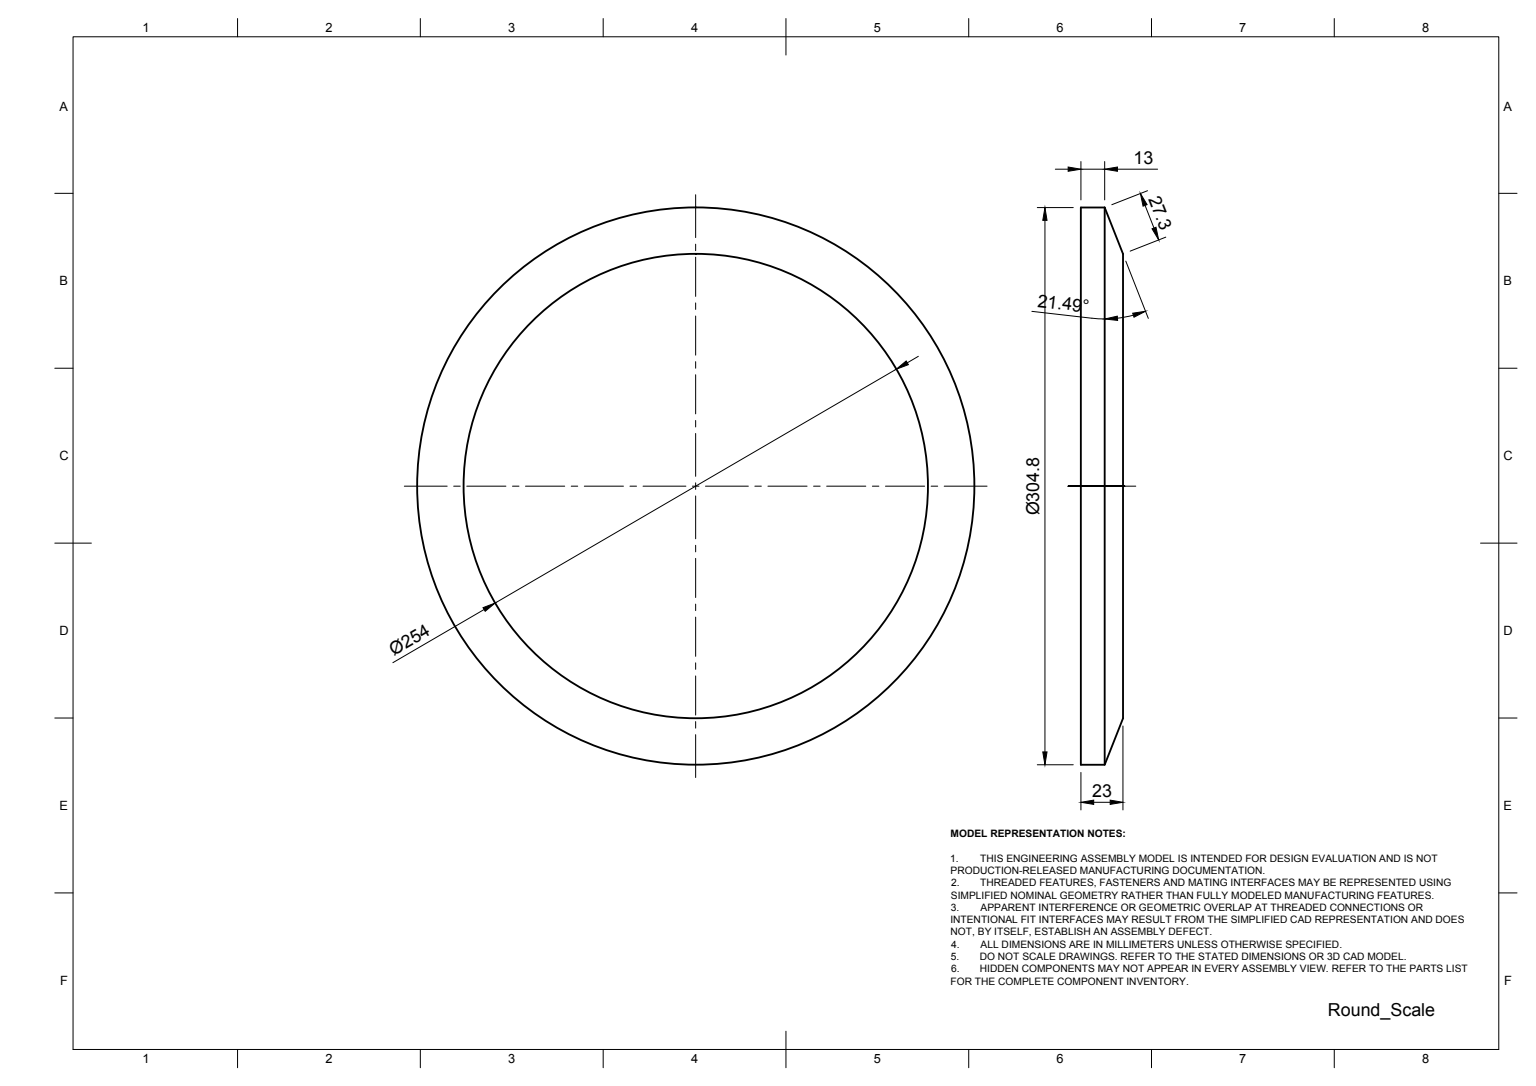
ISO-10303-21;
HEADER;
/* Generated by software containing ST-Developer
 * from STEP Tools, Inc. (www.steptools.com) 
 */

FILE_DESCRIPTION(
/* description */ (''),
/* implementation_level */ '2;1');

FILE_NAME(
/* name */ 'Round_Scale.step',
/* time_stamp */ '2026-10-05T19:45:59-07:00',
/* author */ (''),
/* organization */ (''),
/* preprocessor_version */ 'ST-DEVELOPER v20.2',
/* originating_system */ 'Autodesk Translation Framework v15.15.0.0',
/* authorisation */ '');

FILE_SCHEMA (('AUTOMOTIVE_DESIGN { 1 0 10303 214 3 1 1 }'));
ENDSEC;

DATA;
#10=MECHANICAL_DESIGN_GEOMETRIC_PRESENTATION_REPRESENTATION('',(#95),#2462);
#56=CONICAL_SURFACE('',#1505,139.7,1.19573207282673);
#77=SHAPE_REPRESENTATION_RELATIONSHIP('SRR','None',#2503,#86);
#86=ADVANCED_BREP_SHAPE_REPRESENTATION('',(#104),#2458);
#95=STYLED_ITEM('',(#2552),#104);
#104=MANIFOLD_SOLID_BREP('Body1',#1332);
#134=PLANE('',#1507);
#135=PLANE('',#1508);
#202=FACE_OUTER_BOUND('',#290,.T.);
#203=FACE_OUTER_BOUND('',#291,.T.);
#204=FACE_OUTER_BOUND('',#292,.T.);
#205=FACE_OUTER_BOUND('',#293,.T.);
#290=EDGE_LOOP('',(#1044,#1045,#1046,#1047));
#291=EDGE_LOOP('',(#1048,#1049,#1050,#1051));
#292=EDGE_LOOP('',(#1052));
#293=EDGE_LOOP('',(#1053));
#393=LINE('',#2157,#512);
#394=LINE('',#2161,#513);
#512=VECTOR('',#1768,152.4);
#513=VECTOR('',#1773,139.7);
#600=CIRCLE('',#1503,152.4);
#601=CIRCLE('',#1504,152.4);
#602=CIRCLE('',#1506,127.);
#671=VERTEX_POINT('',#2154);
#672=VERTEX_POINT('',#2156);
#673=VERTEX_POINT('',#2160);
#803=EDGE_CURVE('',#671,#671,#600,.T.);
#804=EDGE_CURVE('',#671,#672,#393,.T.);
#805=EDGE_CURVE('',#672,#672,#601,.F.);
#806=EDGE_CURVE('',#671,#673,#394,.T.);
#807=EDGE_CURVE('',#673,#673,#602,.T.);
#1044=ORIENTED_EDGE('',*,*,#803,.F.);
#1045=ORIENTED_EDGE('',*,*,#804,.T.);
#1046=ORIENTED_EDGE('',*,*,#805,.T.);
#1047=ORIENTED_EDGE('',*,*,#804,.F.);
#1048=ORIENTED_EDGE('',*,*,#803,.T.);
#1049=ORIENTED_EDGE('',*,*,#806,.T.);
#1050=ORIENTED_EDGE('',*,*,#807,.F.);
#1051=ORIENTED_EDGE('',*,*,#806,.F.);
#1052=ORIENTED_EDGE('',*,*,#807,.T.);
#1053=ORIENTED_EDGE('',*,*,#805,.F.);
#1237=CYLINDRICAL_SURFACE('',#1502,152.4);
#1284=ADVANCED_FACE('',(#202),#1237,.T.);
#1285=ADVANCED_FACE('',(#203),#56,.T.);
#1286=ADVANCED_FACE('',(#204),#134,.T.);
#1287=ADVANCED_FACE('',(#205),#135,.T.);
#1332=CLOSED_SHELL('',(#1284,#1285,#1286,#1287));
#1501=AXIS2_PLACEMENT_3D('',#2152,#1762,#1763);
#1502=AXIS2_PLACEMENT_3D('',#2153,#1764,#1765);
#1503=AXIS2_PLACEMENT_3D('',#2155,#1766,#1767);
#1504=AXIS2_PLACEMENT_3D('',#2158,#1769,#1770);
#1505=AXIS2_PLACEMENT_3D('',#2159,#1771,#1772);
#1506=AXIS2_PLACEMENT_3D('',#2162,#1774,#1775);
#1507=AXIS2_PLACEMENT_3D('',#2163,#1776,#1777);
#1508=AXIS2_PLACEMENT_3D('',#2164,#1778,#1779);
#1762=DIRECTION('axis',(0.,0.,1.));
#1763=DIRECTION('refdir',(1.,0.,0.));
#1764=DIRECTION('center_axis',(0.,0.,1.));
#1765=DIRECTION('ref_axis',(1.,0.,0.));
#1766=DIRECTION('center_axis',(0.,0.,1.));
#1767=DIRECTION('ref_axis',(1.,0.,0.));
#1768=DIRECTION('',(0.,0.,-1.));
#1769=DIRECTION('center_axis',(0.,0.,-1.));
#1770=DIRECTION('ref_axis',(1.,0.,0.));
#1771=DIRECTION('center_axis',(0.,0.,-1.));
#1772=DIRECTION('ref_axis',(1.,0.,0.));
#1773=DIRECTION('',(0.930484085528072,-1.13951435699951E-16,0.366332317137032));
#1774=DIRECTION('center_axis',(0.,0.,1.));
#1775=DIRECTION('ref_axis',(1.,0.,0.));
#1776=DIRECTION('center_axis',(0.,0.,1.));
#1777=DIRECTION('ref_axis',(1.,0.,0.));
#1778=DIRECTION('center_axis',(0.,0.,-1.));
#1779=DIRECTION('ref_axis',(-1.,0.,0.));
#2152=CARTESIAN_POINT('',(0.,0.,0.));
#2153=CARTESIAN_POINT('Origin',(-205.724822686805,0.,-24.5));
#2154=CARTESIAN_POINT('',(-358.124822686805,-1.86636172190057E-14,-22.));
#2155=CARTESIAN_POINT('Origin',(-205.724822686805,0.,-22.));
#2156=CARTESIAN_POINT('',(-358.124822686805,1.86636172190057E-14,-35.));
#2157=CARTESIAN_POINT('',(-358.124822686805,-1.86636172190057E-14,-24.5));
#2158=CARTESIAN_POINT('Origin',(-205.724822686805,0.,-35.));
#2159=CARTESIAN_POINT('Origin',(-205.724822686805,0.,-17.));
#2160=CARTESIAN_POINT('',(-332.724822686805,-1.55530143491714E-14,-12.));
#2161=CARTESIAN_POINT('',(-345.424822686805,1.71083157840885E-14,-17.));
#2162=CARTESIAN_POINT('Origin',(-205.724822686805,0.,-12.));
#2163=CARTESIAN_POINT('Origin',(-205.724822686805,0.,-12.));
#2164=CARTESIAN_POINT('Origin',(-53.3248226868051,0.,-35.));
#2447=UNCERTAINTY_MEASURE_WITH_UNIT(LENGTH_MEASURE(0.01),#2463,
'DISTANCE_ACCURACY_VALUE',
'Maximum model space distance between geometric entities at asserted c
onnectivities');
#2451=UNCERTAINTY_MEASURE_WITH_UNIT(LENGTH_MEASURE(0.01),#2463,
'DISTANCE_ACCURACY_VALUE',
'Maximum model space distance between geometric entities at asserted c
onnectivities');
#2458=(
GEOMETRIC_REPRESENTATION_CONTEXT(3)
GLOBAL_UNCERTAINTY_ASSIGNED_CONTEXT((#2447))
GLOBAL_UNIT_ASSIGNED_CONTEXT((#2463,#2465,#2466))
REPRESENTATION_CONTEXT('','3D')
);
#2462=(
GEOMETRIC_REPRESENTATION_CONTEXT(3)
GLOBAL_UNCERTAINTY_ASSIGNED_CONTEXT((#2451))
GLOBAL_UNIT_ASSIGNED_CONTEXT((#2463,#2465,#2466))
REPRESENTATION_CONTEXT('','3D')
);
#2463=(
LENGTH_UNIT()
NAMED_UNIT(*)
SI_UNIT(.MILLI.,.METRE.)
);
#2465=(
NAMED_UNIT(*)
PLANE_ANGLE_UNIT()
SI_UNIT($,.RADIAN.)
);
#2466=(
NAMED_UNIT(*)
SI_UNIT($,.STERADIAN.)
SOLID_ANGLE_UNIT()
);
#2473=SHAPE_DEFINITION_REPRESENTATION(#2483,#2503);
#2483=PRODUCT_DEFINITION_SHAPE('',$,#2514);
#2503=SHAPE_REPRESENTATION('',(#1501),#2458);
#2507=PRODUCT_DEFINITION_CONTEXT('part definition',#2539,'design');
#2514=PRODUCT_DEFINITION('Round_Scale','Round_Scale',#2524,#2507);
#2524=PRODUCT_DEFINITION_FORMATION('',$,#2547);
#2539=APPLICATION_CONTEXT(
'Core Data for Automotive Mechanical Design Process');
#2540=PRODUCT_CONTEXT('part definition',#2539,'mechanical');
#2547=PRODUCT('Round_Scale','Round_Scale',$,(#2540));
#2552=PRESENTATION_STYLE_ASSIGNMENT((#2555));
#2555=SURFACE_STYLE_USAGE(.BOTH.,#2558);
#2558=SURFACE_SIDE_STYLE('',(#2561));
#2561=SURFACE_STYLE_FILL_AREA(#2564);
#2564=FILL_AREA_STYLE('Opaque(160,160,160)',(#2567));
#2567=FILL_AREA_STYLE_COLOUR('Opaque(160,160,160)',#2570);
#2570=COLOUR_RGB('Opaque(160,160,160)', 0.09019608, 0.27058824, 0.51372549);
ENDSEC;
END-ISO-10303-21;
